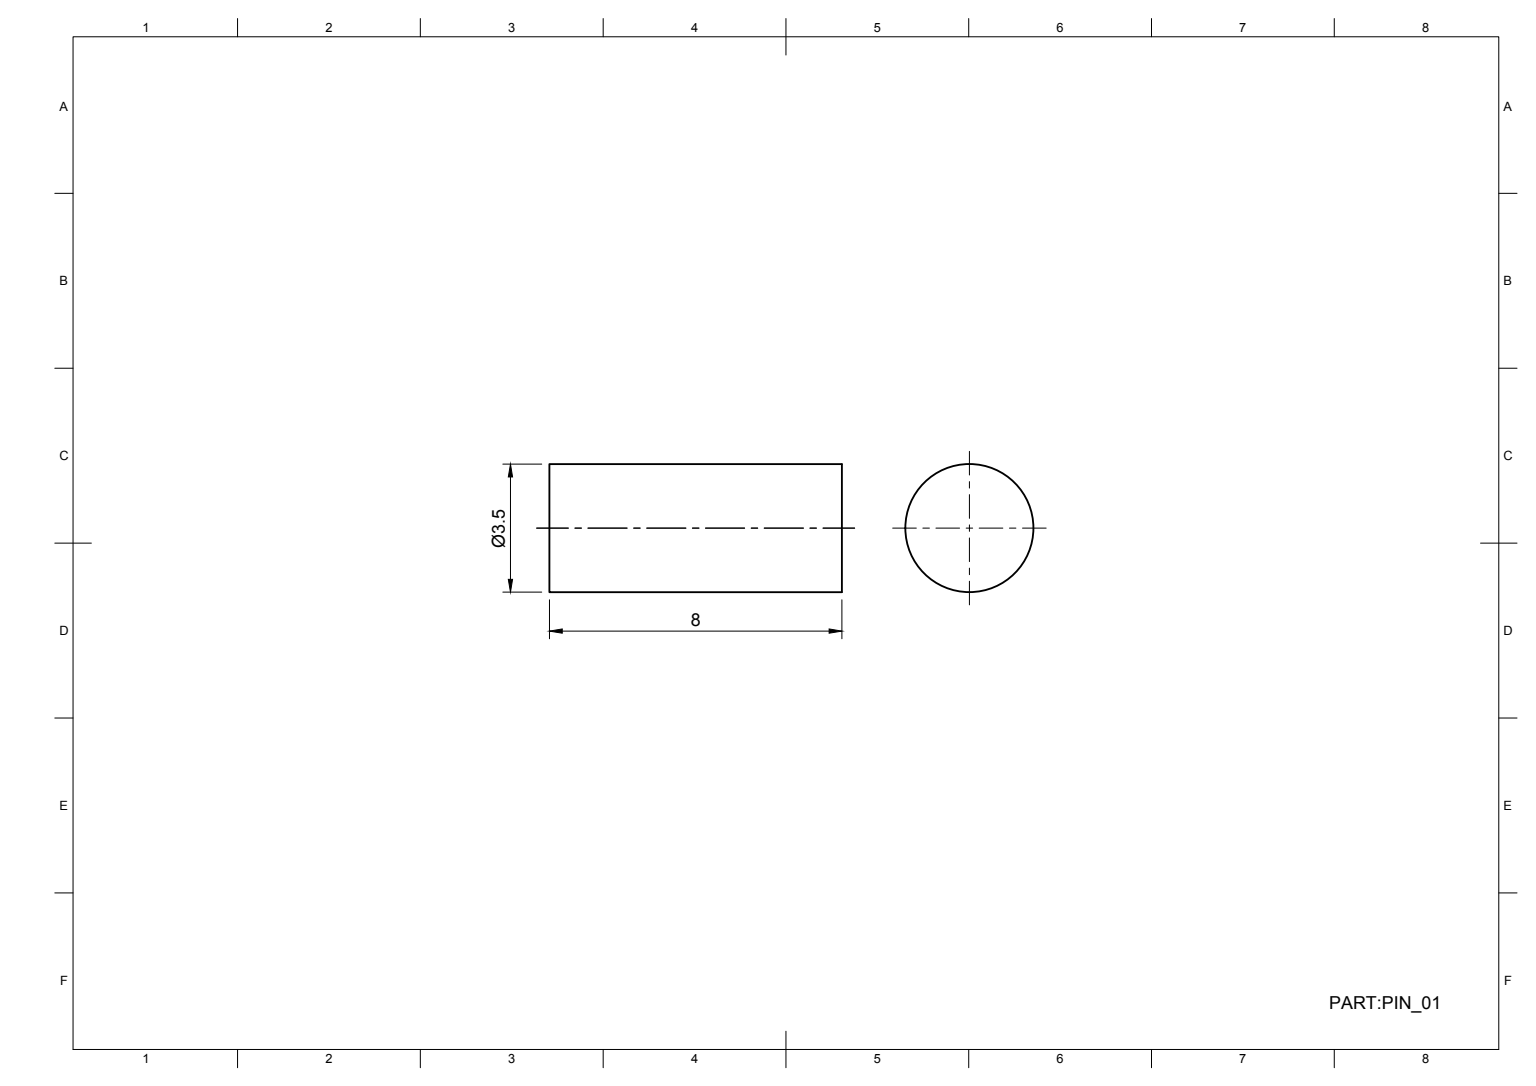
ISO-10303-21;
HEADER;
/* Generated by software containing ST-Developer
 * from STEP Tools, Inc. (www.steptools.com) 
 */

FILE_DESCRIPTION(
/* description */ (''),
/* implementation_level */ '2;1');

FILE_NAME(
/* name */ 'Pin_01.step',
/* time_stamp */ '2026-09-20T21:52:48+06:00',
/* author */ (''),
/* organization */ (''),
/* preprocessor_version */ 'ST-DEVELOPER v20.2',
/* originating_system */ 'Autodesk Translation Framework v15.15.0.0',
/* authorisation */ '');

FILE_SCHEMA (('AUTOMOTIVE_DESIGN { 1 0 10303 214 3 1 1 }'));
ENDSEC;

DATA;
#10=MECHANICAL_DESIGN_GEOMETRIC_PRESENTATION_REPRESENTATION('',(#60),#2203);
#44=SHAPE_REPRESENTATION_RELATIONSHIP('SRR','None',#2236,#52);
#52=ADVANCED_BREP_SHAPE_REPRESENTATION('',(#68),#2196);
#60=STYLED_ITEM('',(#2285),#68);
#68=MANIFOLD_SOLID_BREP('Pin_01',#1227);
#107=CIRCLE('',#1372,1.75);
#108=CIRCLE('',#1374,1.75);
#146=CYLINDRICAL_SURFACE('',#1373,1.75);
#188=FACE_OUTER_BOUND('',#259,.T.);
#189=FACE_OUTER_BOUND('',#260,.T.);
#190=FACE_OUTER_BOUND('',#261,.T.);
#259=EDGE_LOOP('',(#946));
#260=EDGE_LOOP('',(#947,#948,#949,#950));
#261=EDGE_LOOP('',(#951));
#370=LINE('',#1995,#480);
#480=VECTOR('',#1616,1.75);
#583=VERTEX_POINT('',#1991);
#584=VERTEX_POINT('',#1994);
#713=EDGE_CURVE('',#583,#583,#107,.T.);
#714=EDGE_CURVE('',#583,#584,#370,.T.);
#715=EDGE_CURVE('',#584,#584,#108,.T.);
#946=ORIENTED_EDGE('',*,*,#713,.T.);
#947=ORIENTED_EDGE('',*,*,#713,.F.);
#948=ORIENTED_EDGE('',*,*,#714,.T.);
#949=ORIENTED_EDGE('',*,*,#715,.T.);
#950=ORIENTED_EDGE('',*,*,#714,.F.);
#951=ORIENTED_EDGE('',*,*,#715,.F.);
#1130=PLANE('',#1371);
#1131=PLANE('',#1375);
#1184=ADVANCED_FACE('',(#188),#1130,.F.);
#1185=ADVANCED_FACE('',(#189),#146,.T.);
#1186=ADVANCED_FACE('',(#190),#1131,.T.);
#1227=CLOSED_SHELL('',(#1184,#1185,#1186));
#1370=AXIS2_PLACEMENT_3D('',#1989,#1608,#1609);
#1371=AXIS2_PLACEMENT_3D('',#1990,#1610,#1611);
#1372=AXIS2_PLACEMENT_3D('',#1992,#1612,#1613);
#1373=AXIS2_PLACEMENT_3D('',#1993,#1614,#1615);
#1374=AXIS2_PLACEMENT_3D('',#1996,#1617,#1618);
#1375=AXIS2_PLACEMENT_3D('',#1997,#1619,#1620);
#1608=DIRECTION('axis',(0.,0.,1.));
#1609=DIRECTION('refdir',(1.,0.,0.));
#1610=DIRECTION('center_axis',(0.,1.,0.));
#1611=DIRECTION('ref_axis',(1.,0.,0.));
#1612=DIRECTION('center_axis',(0.,-1.,0.));
#1613=DIRECTION('ref_axis',(1.,0.,0.));
#1614=DIRECTION('center_axis',(0.,-1.,0.));
#1615=DIRECTION('ref_axis',(1.,0.,0.));
#1616=DIRECTION('',(0.,1.,0.));
#1617=DIRECTION('center_axis',(0.,-1.,0.));
#1618=DIRECTION('ref_axis',(1.,0.,0.));
#1619=DIRECTION('center_axis',(0.,1.,0.));
#1620=DIRECTION('ref_axis',(1.,0.,0.));
#1989=CARTESIAN_POINT('',(0.,0.,0.));
#1990=CARTESIAN_POINT('Origin',(23.2879869008357,-5.,49.5879869008357));
#1991=CARTESIAN_POINT('',(21.5379869008357,-5.,49.5879869008357));
#1992=CARTESIAN_POINT('Origin',(23.2879869008357,-5.,49.5879869008357));
#1993=CARTESIAN_POINT('Origin',(23.2879869008357,0.,49.5879869008357));
#1994=CARTESIAN_POINT('',(21.5379869008357,3.,49.5879869008357));
#1995=CARTESIAN_POINT('',(21.5379869008357,0.,49.5879869008357));
#1996=CARTESIAN_POINT('Origin',(23.2879869008357,3.,49.5879869008357));
#1997=CARTESIAN_POINT('Origin',(14.3033855617004,3.,40.6033855617004));
#2186=UNCERTAINTY_MEASURE_WITH_UNIT(LENGTH_MEASURE(0.01),#2204,
'DISTANCE_ACCURACY_VALUE',
'Maximum model space distance between geometric entities at asserted c
onnectivities');
#2193=UNCERTAINTY_MEASURE_WITH_UNIT(LENGTH_MEASURE(0.01),#2204,
'DISTANCE_ACCURACY_VALUE',
'Maximum model space distance between geometric entities at asserted c
onnectivities');
#2196=(
GEOMETRIC_REPRESENTATION_CONTEXT(3)
GLOBAL_UNCERTAINTY_ASSIGNED_CONTEXT((#2186))
GLOBAL_UNIT_ASSIGNED_CONTEXT((#2204,#2206,#2207))
REPRESENTATION_CONTEXT('','3D')
);
#2203=(
GEOMETRIC_REPRESENTATION_CONTEXT(3)
GLOBAL_UNCERTAINTY_ASSIGNED_CONTEXT((#2193))
GLOBAL_UNIT_ASSIGNED_CONTEXT((#2204,#2206,#2207))
REPRESENTATION_CONTEXT('','3D')
);
#2204=(
LENGTH_UNIT()
NAMED_UNIT(*)
SI_UNIT(.MILLI.,.METRE.)
);
#2206=(
NAMED_UNIT(*)
PLANE_ANGLE_UNIT()
SI_UNIT($,.RADIAN.)
);
#2207=(
NAMED_UNIT(*)
SI_UNIT($,.STERADIAN.)
SOLID_ANGLE_UNIT()
);
#2210=SHAPE_DEFINITION_REPRESENTATION(#2219,#2236);
#2219=PRODUCT_DEFINITION_SHAPE('',$,#2246);
#2236=SHAPE_REPRESENTATION('',(#1370),#2196);
#2243=PRODUCT_DEFINITION_CONTEXT('part definition',#2272,'design');
#2246=PRODUCT_DEFINITION('Pin_01','Pin_01',#2255,#2243);
#2255=PRODUCT_DEFINITION_FORMATION('',$,#2276);
#2272=APPLICATION_CONTEXT(
'Core Data for Automotive Mechanical Design Process');
#2273=PRODUCT_CONTEXT('part definition',#2272,'mechanical');
#2276=PRODUCT('Pin_01','Pin_01',$,(#2273));
#2285=PRESENTATION_STYLE_ASSIGNMENT((#2289));
#2289=SURFACE_STYLE_USAGE(.BOTH.,#2293);
#2293=SURFACE_SIDE_STYLE('',(#2297));
#2297=SURFACE_STYLE_FILL_AREA(#2301);
#2301=FILL_AREA_STYLE('Surface - Matte',(#2305));
#2305=FILL_AREA_STYLE_COLOUR('Surface - Matte',#2309);
#2309=COLOUR_RGB('Surface - Matte', 0.66274510, 0.83137255, 0.94901961);
ENDSEC;
END-ISO-10303-21;
